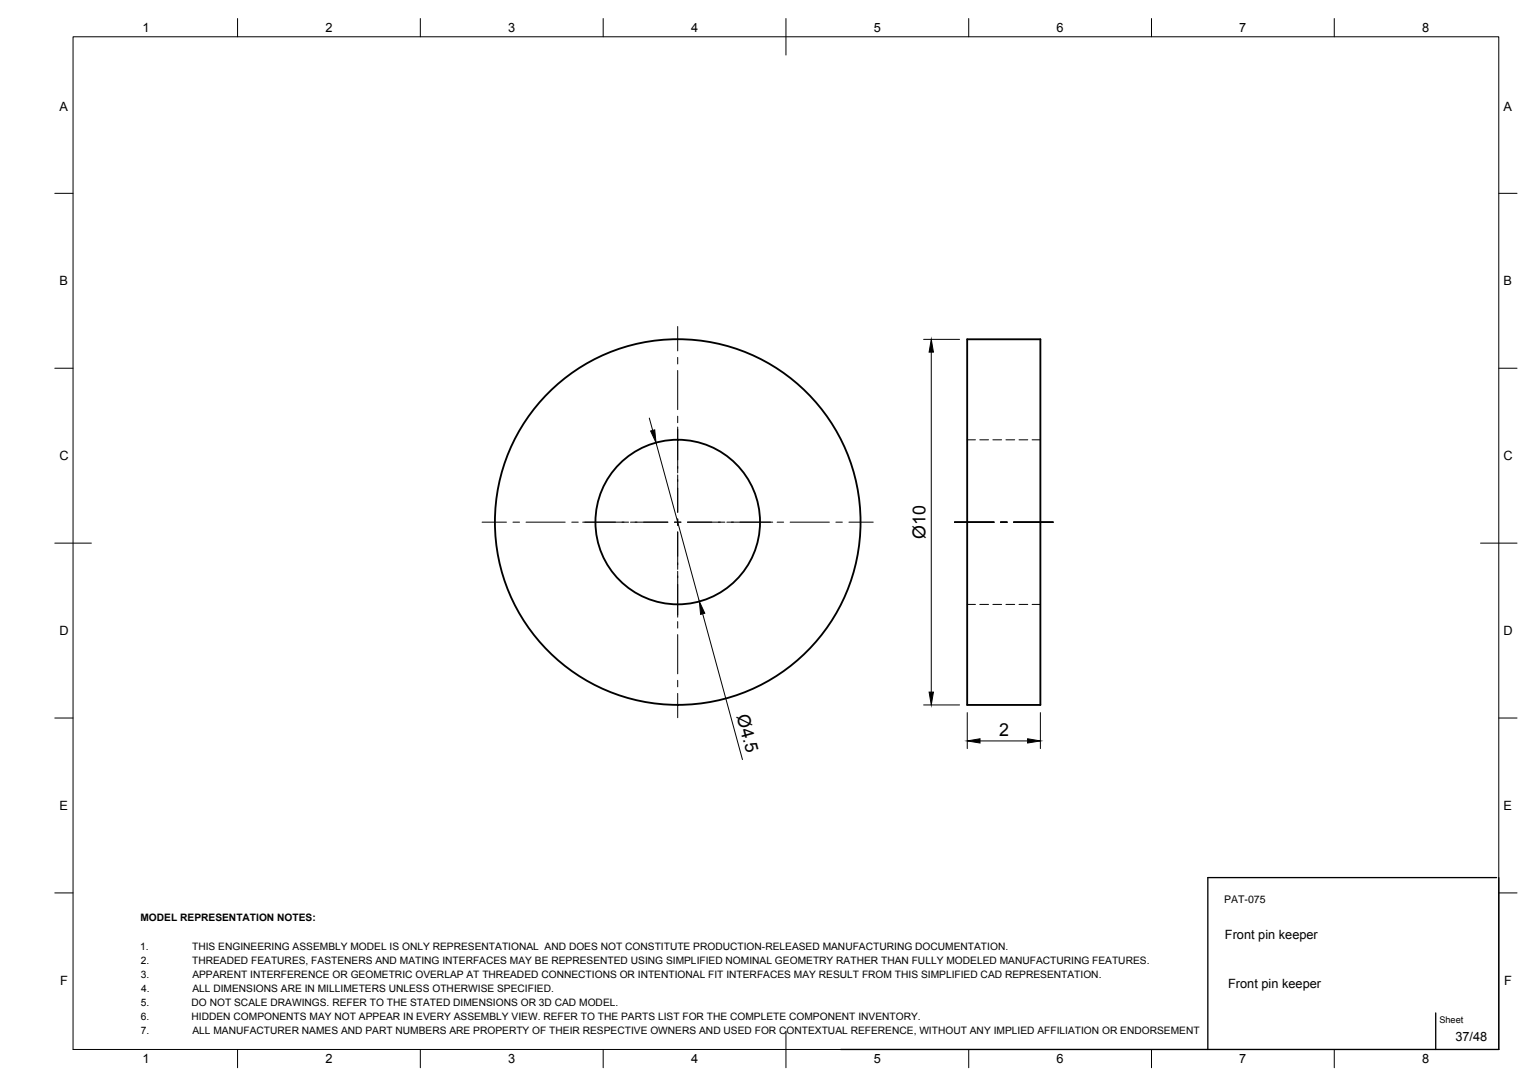
ISO-10303-21;
HEADER;
/* Generated by software containing ST-Developer
 * from STEP Tools, Inc. (www.steptools.com) 
 */

FILE_DESCRIPTION(
/* description */ ('Over-Centre Plunger Toggle Clamp on Slotted Fixture Frame'),
/* implementation_level */ '2;1');

FILE_NAME(
/* name */ 
'Front pin keeper.step',
/* time_stamp */ '2026-10-28T03:23:24-07:00',
/* author */ (''),
/* organization */ (''),
/* preprocessor_version */ 'ST-DEVELOPER v20.2',
/* originating_system */ 'Autodesk Translation Framework v15.17.0.0',
/* authorisation */ '');

FILE_SCHEMA (('AUTOMOTIVE_DESIGN { 1 0 10303 214 3 1 1 }'));
ENDSEC;

DATA;
#10=MECHANICAL_DESIGN_GEOMETRIC_PRESENTATION_REPRESENTATION('',(#551),#15212);
#459=SHAPE_REPRESENTATION_RELATIONSHIP('SRR','None',#15436,#501);
#501=ADVANCED_BREP_SHAPE_REPRESENTATION('',(#600),#15198);
#551=STYLED_ITEM('',(#15719),#600);
#600=MANIFOLD_SOLID_BREP('Body1',#8285);
#761=FACE_BOUND('',#2100,.T.);
#762=FACE_BOUND('',#2102,.T.);
#1011=PLANE('',#9489);
#1012=PLANE('',#9490);
#1461=FACE_OUTER_BOUND('',#2097,.T.);
#1462=FACE_OUTER_BOUND('',#2098,.T.);
#1463=FACE_OUTER_BOUND('',#2099,.T.);
#1464=FACE_OUTER_BOUND('',#2101,.T.);
#2097=EDGE_LOOP('',(#7183,#7184,#7185,#7186));
#2098=EDGE_LOOP('',(#7187,#7188,#7189,#7190));
#2099=EDGE_LOOP('',(#7191));
#2100=EDGE_LOOP('',(#7192));
#2101=EDGE_LOOP('',(#7193));
#2102=EDGE_LOOP('',(#7194));
#2713=LINE('',#14537,#3343);
#2714=LINE('',#14543,#3344);
#3343=VECTOR('',#11680,0.225);
#3344=VECTOR('',#11687,0.5);
#3792=CIRCLE('',#9484,0.225);
#3793=CIRCLE('',#9485,0.225);
#3794=CIRCLE('',#9487,0.5);
#3795=CIRCLE('',#9488,0.5);
#4404=VERTEX_POINT('',#14534);
#4405=VERTEX_POINT('',#14536);
#4406=VERTEX_POINT('',#14540);
#4407=VERTEX_POINT('',#14542);
#5352=EDGE_CURVE('',#4404,#4404,#3792,.T.);
#5353=EDGE_CURVE('',#4404,#4405,#2713,.T.);
#5354=EDGE_CURVE('',#4405,#4405,#3793,.T.);
#5355=EDGE_CURVE('',#4406,#4406,#3794,.T.);
#5356=EDGE_CURVE('',#4406,#4407,#2714,.T.);
#5357=EDGE_CURVE('',#4407,#4407,#3795,.T.);
#7183=ORIENTED_EDGE('',*,*,#5352,.F.);
#7184=ORIENTED_EDGE('',*,*,#5353,.T.);
#7185=ORIENTED_EDGE('',*,*,#5354,.T.);
#7186=ORIENTED_EDGE('',*,*,#5353,.F.);
#7187=ORIENTED_EDGE('',*,*,#5355,.F.);
#7188=ORIENTED_EDGE('',*,*,#5356,.T.);
#7189=ORIENTED_EDGE('',*,*,#5357,.T.);
#7190=ORIENTED_EDGE('',*,*,#5356,.F.);
#7191=ORIENTED_EDGE('',*,*,#5355,.T.);
#7192=ORIENTED_EDGE('',*,*,#5352,.T.);
#7193=ORIENTED_EDGE('',*,*,#5357,.F.);
#7194=ORIENTED_EDGE('',*,*,#5354,.F.);
#7733=CYLINDRICAL_SURFACE('',#9483,0.225);
#7734=CYLINDRICAL_SURFACE('',#9486,0.5);
#8133=ADVANCED_FACE('',(#1461),#7733,.F.);
#8134=ADVANCED_FACE('',(#1462),#7734,.T.);
#8135=ADVANCED_FACE('',(#1463,#761),#1011,.T.);
#8136=ADVANCED_FACE('',(#1464,#762),#1012,.F.);
#8285=CLOSED_SHELL('',(#8133,#8134,#8135,#8136));
#9482=AXIS2_PLACEMENT_3D('',#14532,#11674,#11675);
#9483=AXIS2_PLACEMENT_3D('',#14533,#11676,#11677);
#9484=AXIS2_PLACEMENT_3D('',#14535,#11678,#11679);
#9485=AXIS2_PLACEMENT_3D('',#14538,#11681,#11682);
#9486=AXIS2_PLACEMENT_3D('',#14539,#11683,#11684);
#9487=AXIS2_PLACEMENT_3D('',#14541,#11685,#11686);
#9488=AXIS2_PLACEMENT_3D('',#14544,#11688,#11689);
#9489=AXIS2_PLACEMENT_3D('',#14545,#11690,#11691);
#9490=AXIS2_PLACEMENT_3D('',#14546,#11692,#11693);
#11674=DIRECTION('axis',(0.,0.,1.));
#11675=DIRECTION('refdir',(1.,0.,0.));
#11676=DIRECTION('center_axis',(0.,1.,0.));
#11677=DIRECTION('ref_axis',(1.,0.,0.));
#11678=DIRECTION('center_axis',(0.,-1.,0.));
#11679=DIRECTION('ref_axis',(1.,0.,0.));
#11680=DIRECTION('',(0.,-1.,0.));
#11681=DIRECTION('center_axis',(0.,-1.,0.));
#11682=DIRECTION('ref_axis',(1.,0.,0.));
#11683=DIRECTION('center_axis',(0.,1.,0.));
#11684=DIRECTION('ref_axis',(1.,0.,0.));
#11685=DIRECTION('center_axis',(0.,1.,0.));
#11686=DIRECTION('ref_axis',(1.,0.,0.));
#11687=DIRECTION('',(0.,-1.,0.));
#11688=DIRECTION('center_axis',(0.,1.,0.));
#11689=DIRECTION('ref_axis',(1.,0.,0.));
#11690=DIRECTION('center_axis',(0.,1.,0.));
#11691=DIRECTION('ref_axis',(1.,0.,0.));
#11692=DIRECTION('center_axis',(0.,1.,0.));
#11693=DIRECTION('ref_axis',(1.,0.,0.));
#14532=CARTESIAN_POINT('',(0.,0.,0.));
#14533=CARTESIAN_POINT('Origin',(-2.82632109303527,-5.9,8.79263101785268));
#14534=CARTESIAN_POINT('',(-3.05132109303527,-5.7,8.79263101785268));
#14535=CARTESIAN_POINT('Origin',(-2.82632109303527,-5.7,8.79263101785268));
#14536=CARTESIAN_POINT('',(-3.05132109303527,-5.9,8.79263101785268));
#14537=CARTESIAN_POINT('',(-3.05132109303527,-5.9,8.79263101785268));
#14538=CARTESIAN_POINT('Origin',(-2.82632109303527,-5.9,8.79263101785268));
#14539=CARTESIAN_POINT('Origin',(-2.82632109303527,-5.9,8.79263101785268));
#14540=CARTESIAN_POINT('',(-3.32632109303527,-5.7,8.79263101785268));
#14541=CARTESIAN_POINT('Origin',(-2.82632109303527,-5.7,8.79263101785268));
#14542=CARTESIAN_POINT('',(-3.32632109303527,-5.9,8.79263101785268));
#14543=CARTESIAN_POINT('',(-3.32632109303527,-5.9,8.79263101785268));
#14544=CARTESIAN_POINT('Origin',(-2.82632109303527,-5.9,8.79263101785268));
#14545=CARTESIAN_POINT('Origin',(-2.82632109303527,-5.7,8.79263101785268));
#14546=CARTESIAN_POINT('Origin',(-2.82632109303527,-5.9,8.79263101785268));
#15148=UNCERTAINTY_MEASURE_WITH_UNIT(LENGTH_MEASURE(0.001),#15213,
'DISTANCE_ACCURACY_VALUE',
'Maximum model space distance between geometric entities at asserted c
onnectivities');
#15162=UNCERTAINTY_MEASURE_WITH_UNIT(LENGTH_MEASURE(0.001),#15213,
'DISTANCE_ACCURACY_VALUE',
'Maximum model space distance between geometric entities at asserted c
onnectivities');
#15198=(
GEOMETRIC_REPRESENTATION_CONTEXT(3)
GLOBAL_UNCERTAINTY_ASSIGNED_CONTEXT((#15148))
GLOBAL_UNIT_ASSIGNED_CONTEXT((#15213,#15215,#15216))
REPRESENTATION_CONTEXT('','3D')
);
#15212=(
GEOMETRIC_REPRESENTATION_CONTEXT(3)
GLOBAL_UNCERTAINTY_ASSIGNED_CONTEXT((#15162))
GLOBAL_UNIT_ASSIGNED_CONTEXT((#15213,#15215,#15216))
REPRESENTATION_CONTEXT('','3D')
);
#15213=(
LENGTH_UNIT()
NAMED_UNIT(*)
SI_UNIT(.CENTI.,.METRE.)
);
#15215=(
NAMED_UNIT(*)
PLANE_ANGLE_UNIT()
SI_UNIT($,.RADIAN.)
);
#15216=(
NAMED_UNIT(*)
SI_UNIT($,.STERADIAN.)
SOLID_ANGLE_UNIT()
);
#15252=SHAPE_DEFINITION_REPRESENTATION(#15308,#15436);
#15308=PRODUCT_DEFINITION_SHAPE('',$,#15486);
#15436=SHAPE_REPRESENTATION('',(#9482),#15198);
#15450=PRODUCT_DEFINITION_CONTEXT('part definition',#15599,'design');
#15486=PRODUCT_DEFINITION('Front pin keeper','Front pin keeper',#15535,
#15450);
#15535=PRODUCT_DEFINITION_FORMATION('',$,#15636);
#15599=APPLICATION_CONTEXT(
'Core Data for Automotive Mechanical Design Process');
#15600=PRODUCT_CONTEXT('part definition',#15599,'mechanical');
#15636=PRODUCT('Front pin keeper','Front pin keeper','Front pin keeper',
(#15600));
#15713=COLOUR_RGB('Grey',0.48,0.52,0.57);
#15714=FILL_AREA_STYLE_COLOUR('',#15713);
#15715=FILL_AREA_STYLE('',(#15714));
#15716=SURFACE_STYLE_FILL_AREA(#15715);
#15717=SURFACE_SIDE_STYLE('',(#15716));
#15718=SURFACE_STYLE_USAGE(.BOTH.,#15717);
#15719=PRESENTATION_STYLE_ASSIGNMENT((#15718));
ENDSEC;
END-ISO-10303-21;
